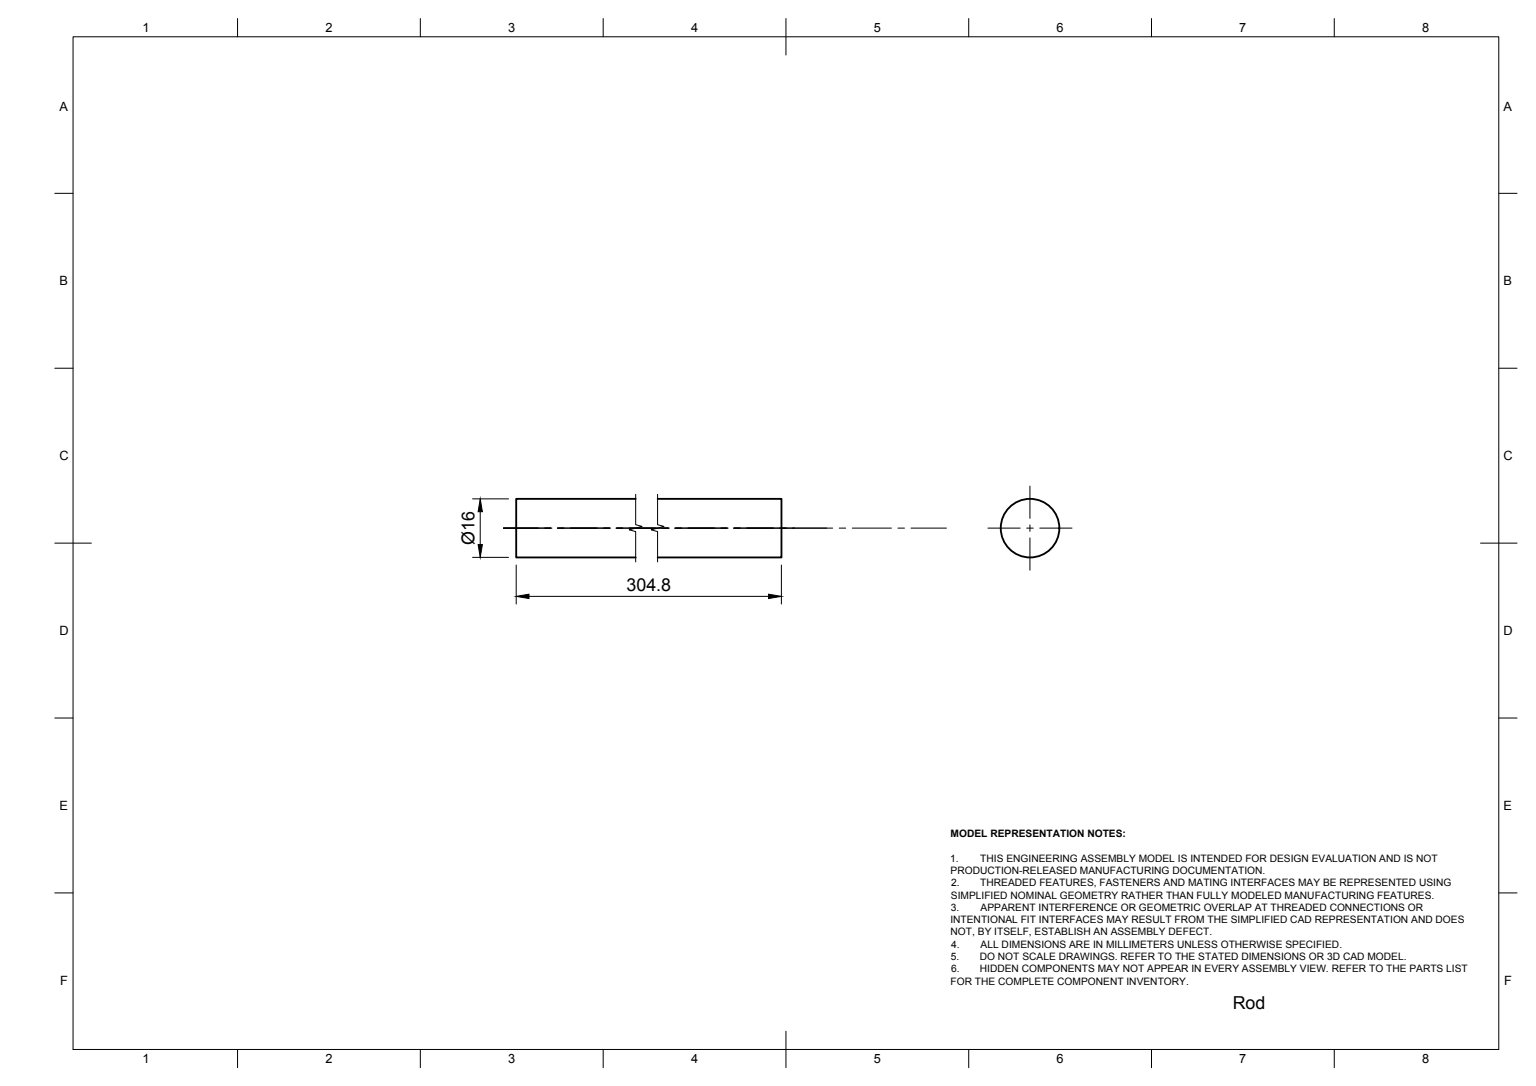
ISO-10303-21;
HEADER;
/* Generated by software containing ST-Developer
 * from STEP Tools, Inc. (www.steptools.com) 
 */

FILE_DESCRIPTION(
/* description */ (''),
/* implementation_level */ '2;1');

FILE_NAME(
/* name */ 'Rod.step',
/* time_stamp */ '2026-10-05T19:45:59-07:00',
/* author */ (''),
/* organization */ (''),
/* preprocessor_version */ 'ST-DEVELOPER v20.2',
/* originating_system */ 'Autodesk Translation Framework v15.15.0.0',
/* authorisation */ '');

FILE_SCHEMA (('AUTOMOTIVE_DESIGN { 1 0 10303 214 3 1 1 }'));
ENDSEC;

DATA;
#10=MECHANICAL_DESIGN_GEOMETRIC_PRESENTATION_REPRESENTATION('',(#90),#2462);
#72=SHAPE_REPRESENTATION_RELATIONSHIP('SRR','None',#2498,#81);
#81=ADVANCED_BREP_SHAPE_REPRESENTATION('',(#99),#2453);
#90=STYLED_ITEM('',(#2552),#99);
#99=MANIFOLD_SOLID_BREP('Body1',#1327);
#108=PLANE('',#1441);
#109=PLANE('',#1442);
#165=FACE_OUTER_BOUND('',#245,.T.);
#166=FACE_OUTER_BOUND('',#246,.T.);
#167=FACE_OUTER_BOUND('',#247,.T.);
#245=EDGE_LOOP('',(#894,#895,#896,#897));
#246=EDGE_LOOP('',(#898));
#247=EDGE_LOOP('',(#899));
#340=LINE('',#1990,#459);
#459=VECTOR('',#1587,8.);
#578=CIRCLE('',#1439,8.);
#579=CIRCLE('',#1440,8.);
#621=VERTEX_POINT('',#1987);
#622=VERTEX_POINT('',#1989);
#728=EDGE_CURVE('',#621,#621,#578,.T.);
#729=EDGE_CURVE('',#621,#622,#340,.T.);
#730=EDGE_CURVE('',#622,#622,#579,.T.);
#894=ORIENTED_EDGE('',*,*,#728,.F.);
#895=ORIENTED_EDGE('',*,*,#729,.T.);
#896=ORIENTED_EDGE('',*,*,#730,.T.);
#897=ORIENTED_EDGE('',*,*,#729,.F.);
#898=ORIENTED_EDGE('',*,*,#728,.T.);
#899=ORIENTED_EDGE('',*,*,#730,.F.);
#1226=CYLINDRICAL_SURFACE('',#1438,8.);
#1247=ADVANCED_FACE('',(#165),#1226,.T.);
#1248=ADVANCED_FACE('',(#166),#108,.T.);
#1249=ADVANCED_FACE('',(#167),#109,.F.);
#1327=CLOSED_SHELL('',(#1247,#1248,#1249));
#1437=AXIS2_PLACEMENT_3D('',#1985,#1581,#1582);
#1438=AXIS2_PLACEMENT_3D('',#1986,#1583,#1584);
#1439=AXIS2_PLACEMENT_3D('',#1988,#1585,#1586);
#1440=AXIS2_PLACEMENT_3D('',#1991,#1588,#1589);
#1441=AXIS2_PLACEMENT_3D('',#1992,#1590,#1591);
#1442=AXIS2_PLACEMENT_3D('',#1993,#1592,#1593);
#1581=DIRECTION('axis',(0.,0.,1.));
#1582=DIRECTION('refdir',(1.,0.,0.));
#1583=DIRECTION('center_axis',(1.,0.,0.));
#1584=DIRECTION('ref_axis',(0.,1.,0.));
#1585=DIRECTION('center_axis',(1.,0.,0.));
#1586=DIRECTION('ref_axis',(0.,1.,0.));
#1587=DIRECTION('',(-1.,0.,0.));
#1588=DIRECTION('center_axis',(1.,0.,0.));
#1589=DIRECTION('ref_axis',(0.,1.,0.));
#1590=DIRECTION('center_axis',(1.,0.,0.));
#1591=DIRECTION('ref_axis',(0.,0.,-1.));
#1592=DIRECTION('center_axis',(1.,0.,0.));
#1593=DIRECTION('ref_axis',(0.,0.,-1.));
#1985=CARTESIAN_POINT('',(0.,0.,0.));
#1986=CARTESIAN_POINT('Origin',(0.,0.,0.));
#1987=CARTESIAN_POINT('',(304.8,-8.,-9.79717439317883E-16));
#1988=CARTESIAN_POINT('Origin',(304.8,0.,0.));
#1989=CARTESIAN_POINT('',(0.,-8.,-9.79717439317883E-16));
#1990=CARTESIAN_POINT('',(0.,-8.,-9.79717439317883E-16));
#1991=CARTESIAN_POINT('Origin',(0.,0.,0.));
#1992=CARTESIAN_POINT('Origin',(304.8,0.,0.));
#1993=CARTESIAN_POINT('Origin',(0.,0.,0.));
#2442=UNCERTAINTY_MEASURE_WITH_UNIT(LENGTH_MEASURE(0.01),#2463,
'DISTANCE_ACCURACY_VALUE',
'Maximum model space distance between geometric entities at asserted c
onnectivities');
#2451=UNCERTAINTY_MEASURE_WITH_UNIT(LENGTH_MEASURE(0.01),#2463,
'DISTANCE_ACCURACY_VALUE',
'Maximum model space distance between geometric entities at asserted c
onnectivities');
#2453=(
GEOMETRIC_REPRESENTATION_CONTEXT(3)
GLOBAL_UNCERTAINTY_ASSIGNED_CONTEXT((#2442))
GLOBAL_UNIT_ASSIGNED_CONTEXT((#2463,#2465,#2466))
REPRESENTATION_CONTEXT('','3D')
);
#2462=(
GEOMETRIC_REPRESENTATION_CONTEXT(3)
GLOBAL_UNCERTAINTY_ASSIGNED_CONTEXT((#2451))
GLOBAL_UNIT_ASSIGNED_CONTEXT((#2463,#2465,#2466))
REPRESENTATION_CONTEXT('','3D')
);
#2463=(
LENGTH_UNIT()
NAMED_UNIT(*)
SI_UNIT(.MILLI.,.METRE.)
);
#2465=(
NAMED_UNIT(*)
PLANE_ANGLE_UNIT()
SI_UNIT($,.RADIAN.)
);
#2466=(
NAMED_UNIT(*)
SI_UNIT($,.STERADIAN.)
SOLID_ANGLE_UNIT()
);
#2468=SHAPE_DEFINITION_REPRESENTATION(#2478,#2498);
#2478=PRODUCT_DEFINITION_SHAPE('',$,#2509);
#2498=SHAPE_REPRESENTATION('',(#1437),#2453);
#2507=PRODUCT_DEFINITION_CONTEXT('part definition',#2539,'design');
#2509=PRODUCT_DEFINITION('Rod','Rod',#2519,#2507);
#2519=PRODUCT_DEFINITION_FORMATION('',$,#2542);
#2539=APPLICATION_CONTEXT(
'Core Data for Automotive Mechanical Design Process');
#2540=PRODUCT_CONTEXT('part definition',#2539,'mechanical');
#2542=PRODUCT('Rod','Rod',$,(#2540));
#2552=PRESENTATION_STYLE_ASSIGNMENT((#2555));
#2555=SURFACE_STYLE_USAGE(.BOTH.,#2558);
#2558=SURFACE_SIDE_STYLE('',(#2561));
#2561=SURFACE_STYLE_FILL_AREA(#2564);
#2564=FILL_AREA_STYLE('Opaque(160,160,160)',(#2567));
#2567=FILL_AREA_STYLE_COLOUR('Opaque(160,160,160)',#2570);
#2570=COLOUR_RGB('Opaque(160,160,160)', 0.09019608, 0.27058824, 0.51372549);
ENDSEC;
END-ISO-10303-21;
